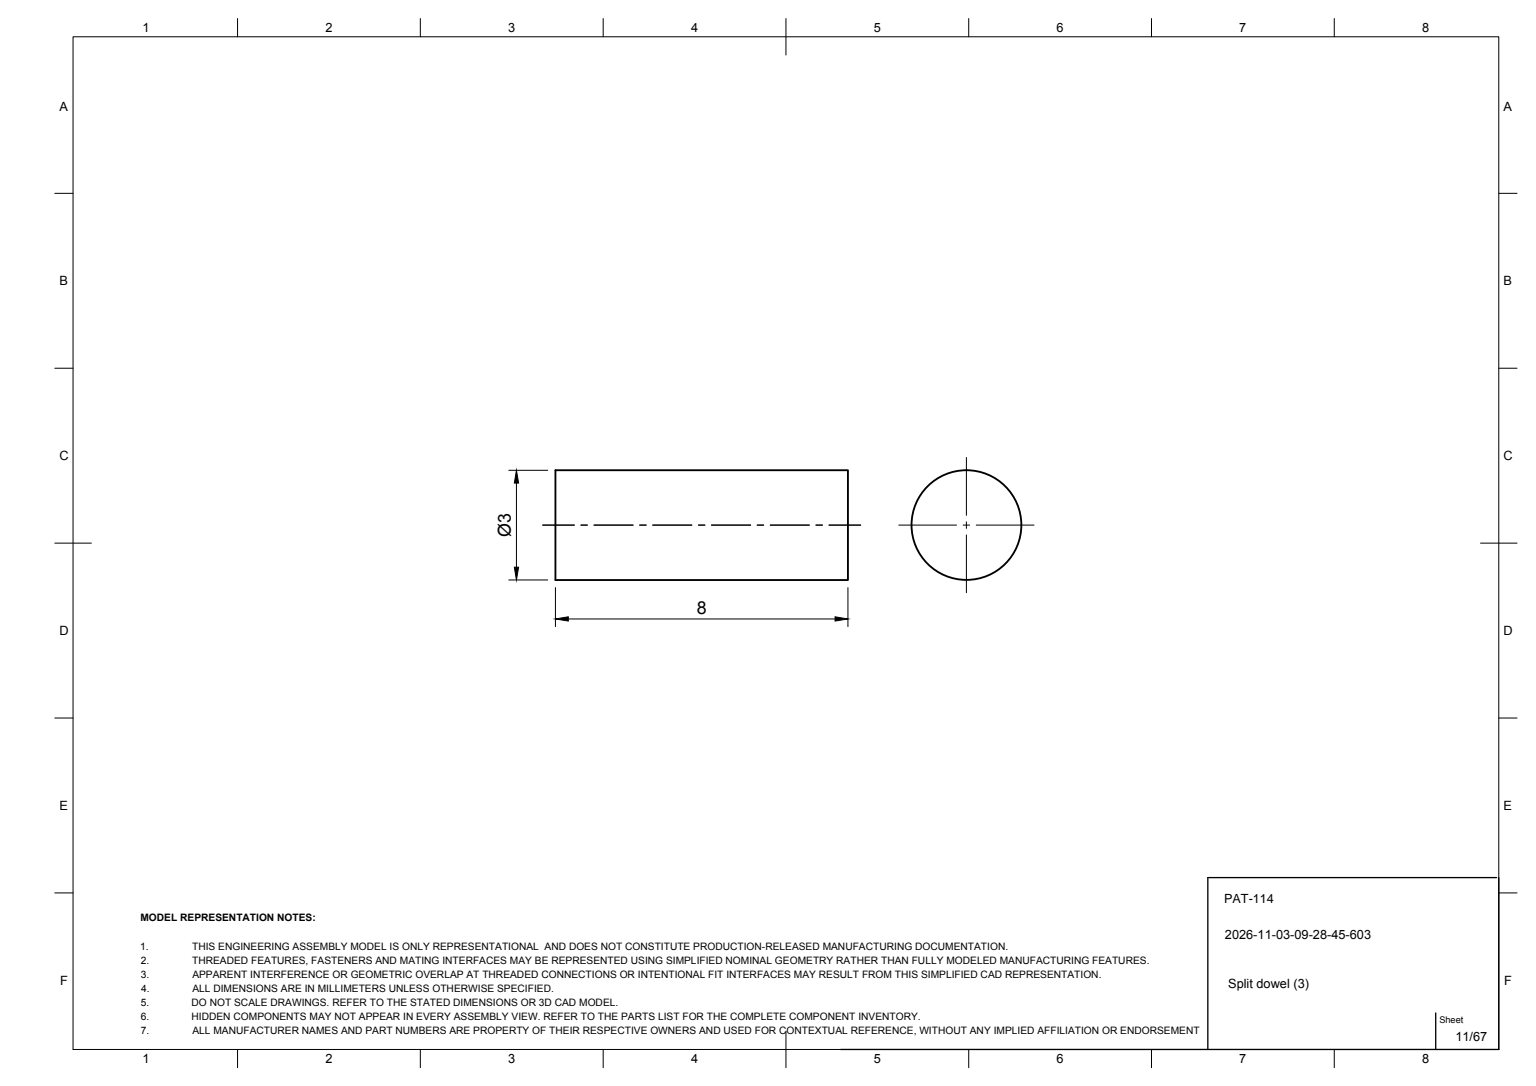
ISO-10303-21;
HEADER;
/* Generated by software containing ST-Developer
 * from STEP Tools, Inc. (www.steptools.com) 
 */

FILE_DESCRIPTION(
/* description */ ('Two-stage gear reducer in split housing'),
/* implementation_level */ '2;1');

FILE_NAME(
/* name */ 'Split dowel (3).step',
/* time_stamp */ '2026-10-28T03:22:31-07:00',
/* author */ (''),
/* organization */ (''),
/* preprocessor_version */ 'ST-DEVELOPER v20.2',
/* originating_system */ 'Autodesk Translation Framework v15.17.0.0',
/* authorisation */ '');

FILE_SCHEMA (('AUTOMOTIVE_DESIGN { 1 0 10303 214 3 1 1 }'));
ENDSEC;

DATA;
#10=MECHANICAL_DESIGN_GEOMETRIC_PRESENTATION_REPRESENTATION('',(#1240),#73366);
#1128=SHAPE_REPRESENTATION_RELATIONSHIP('SRR','None',#73615,#1184);
#1184=ADVANCED_BREP_SHAPE_REPRESENTATION('',(#1311),#73311);
#1240=STYLED_ITEM('',(#73974),#1311);
#1311=MANIFOLD_SOLID_BREP('Body1',#16128);
#1706=PLANE('',#17189);
#1707=PLANE('',#17190);
#2193=FACE_OUTER_BOUND('',#3192,.T.);
#2194=FACE_OUTER_BOUND('',#3193,.T.);
#2195=FACE_OUTER_BOUND('',#3194,.T.);
#3192=EDGE_LOOP('',(#11365,#11366,#11367,#11368));
#3193=EDGE_LOOP('',(#11369));
#3194=EDGE_LOOP('',(#11370));
#4311=LINE('',#23693,#5335);
#5335=VECTOR('',#19465,0.149999999999999);
#6278=CIRCLE('',#17187,0.149999999999999);
#6279=CIRCLE('',#17188,0.149999999999999);
#7110=VERTEX_POINT('',#23690);
#7111=VERTEX_POINT('',#23692);
#8736=EDGE_CURVE('',#7110,#7110,#6278,.T.);
#8737=EDGE_CURVE('',#7110,#7111,#4311,.T.);
#8738=EDGE_CURVE('',#7111,#7111,#6279,.T.);
#11365=ORIENTED_EDGE('',*,*,#8736,.F.);
#11366=ORIENTED_EDGE('',*,*,#8737,.T.);
#11367=ORIENTED_EDGE('',*,*,#8738,.T.);
#11368=ORIENTED_EDGE('',*,*,#8737,.F.);
#11369=ORIENTED_EDGE('',*,*,#8736,.T.);
#11370=ORIENTED_EDGE('',*,*,#8738,.F.);
#14994=CYLINDRICAL_SURFACE('',#17186,0.149999999999999);
#15400=ADVANCED_FACE('',(#2193),#14994,.T.);
#15401=ADVANCED_FACE('',(#2194),#1706,.T.);
#15402=ADVANCED_FACE('',(#2195),#1707,.F.);
#16128=CLOSED_SHELL('',(#15400,#15401,#15402));
#17185=AXIS2_PLACEMENT_3D('',#23688,#19459,#19460);
#17186=AXIS2_PLACEMENT_3D('',#23689,#19461,#19462);
#17187=AXIS2_PLACEMENT_3D('',#23691,#19463,#19464);
#17188=AXIS2_PLACEMENT_3D('',#23694,#19466,#19467);
#17189=AXIS2_PLACEMENT_3D('',#23695,#19468,#19469);
#17190=AXIS2_PLACEMENT_3D('',#23696,#19470,#19471);
#19459=DIRECTION('axis',(0.,0.,1.));
#19460=DIRECTION('refdir',(1.,0.,0.));
#19461=DIRECTION('center_axis',(0.,0.,1.));
#19462=DIRECTION('ref_axis',(1.,0.,0.));
#19463=DIRECTION('center_axis',(0.,0.,1.));
#19464=DIRECTION('ref_axis',(1.,0.,0.));
#19465=DIRECTION('',(0.,0.,-1.));
#19466=DIRECTION('center_axis',(0.,0.,1.));
#19467=DIRECTION('ref_axis',(1.,0.,0.));
#19468=DIRECTION('center_axis',(0.,0.,1.));
#19469=DIRECTION('ref_axis',(1.,0.,0.));
#19470=DIRECTION('center_axis',(0.,0.,1.));
#19471=DIRECTION('ref_axis',(1.,0.,0.));
#23688=CARTESIAN_POINT('',(0.,0.,0.));
#23689=CARTESIAN_POINT('Origin',(17.75,3.,9.6));
#23690=CARTESIAN_POINT('',(17.6,3.,10.4));
#23691=CARTESIAN_POINT('Origin',(17.75,3.,10.4));
#23692=CARTESIAN_POINT('',(17.6,3.,9.6));
#23693=CARTESIAN_POINT('',(17.6,3.,9.6));
#23694=CARTESIAN_POINT('Origin',(17.75,3.,9.6));
#23695=CARTESIAN_POINT('Origin',(17.75,3.,10.4));
#23696=CARTESIAN_POINT('Origin',(17.75,3.,9.6));
#73247=UNCERTAINTY_MEASURE_WITH_UNIT(LENGTH_MEASURE(0.001),#73367,
'DISTANCE_ACCURACY_VALUE',
'Maximum model space distance between geometric entities at asserted c
onnectivities');
#73302=UNCERTAINTY_MEASURE_WITH_UNIT(LENGTH_MEASURE(0.001),#73367,
'DISTANCE_ACCURACY_VALUE',
'Maximum model space distance between geometric entities at asserted c
onnectivities');
#73311=(
GEOMETRIC_REPRESENTATION_CONTEXT(3)
GLOBAL_UNCERTAINTY_ASSIGNED_CONTEXT((#73247))
GLOBAL_UNIT_ASSIGNED_CONTEXT((#73367,#73369,#73370))
REPRESENTATION_CONTEXT('','3D')
);
#73366=(
GEOMETRIC_REPRESENTATION_CONTEXT(3)
GLOBAL_UNCERTAINTY_ASSIGNED_CONTEXT((#73302))
GLOBAL_UNIT_ASSIGNED_CONTEXT((#73367,#73369,#73370))
REPRESENTATION_CONTEXT('','3D')
);
#73367=(
LENGTH_UNIT()
NAMED_UNIT(*)
SI_UNIT(.CENTI.,.METRE.)
);
#73369=(
NAMED_UNIT(*)
PLANE_ANGLE_UNIT()
SI_UNIT($,.RADIAN.)
);
#73370=(
NAMED_UNIT(*)
SI_UNIT($,.STERADIAN.)
SOLID_ANGLE_UNIT()
);
#73379=SHAPE_DEFINITION_REPRESENTATION(#73442,#73615);
#73442=PRODUCT_DEFINITION_SHAPE('',$,#73679);
#73615=SHAPE_REPRESENTATION('',(#17185),#73311);
#73670=PRODUCT_DEFINITION_CONTEXT('part definition',#73861,'design');
#73679=PRODUCT_DEFINITION('Split dowel (3)','Split dowel (3)',#73742,#73670);
#73742=PRODUCT_DEFINITION_FORMATION('',$,#73871);
#73861=APPLICATION_CONTEXT(
'Core Data for Automotive Mechanical Design Process');
#73862=PRODUCT_CONTEXT('part definition',#73861,'mechanical');
#73871=PRODUCT('Split dowel (3)','Split dowel (3)','Split dowel (3)',(#73862));
#73968=COLOUR_RGB('Light Blue',0.38,0.62,0.78);
#73969=FILL_AREA_STYLE_COLOUR('',#73968);
#73970=FILL_AREA_STYLE('',(#73969));
#73971=SURFACE_STYLE_FILL_AREA(#73970);
#73972=SURFACE_SIDE_STYLE('',(#73971));
#73973=SURFACE_STYLE_USAGE(.BOTH.,#73972);
#73974=PRESENTATION_STYLE_ASSIGNMENT((#73973));
ENDSEC;
END-ISO-10303-21;
